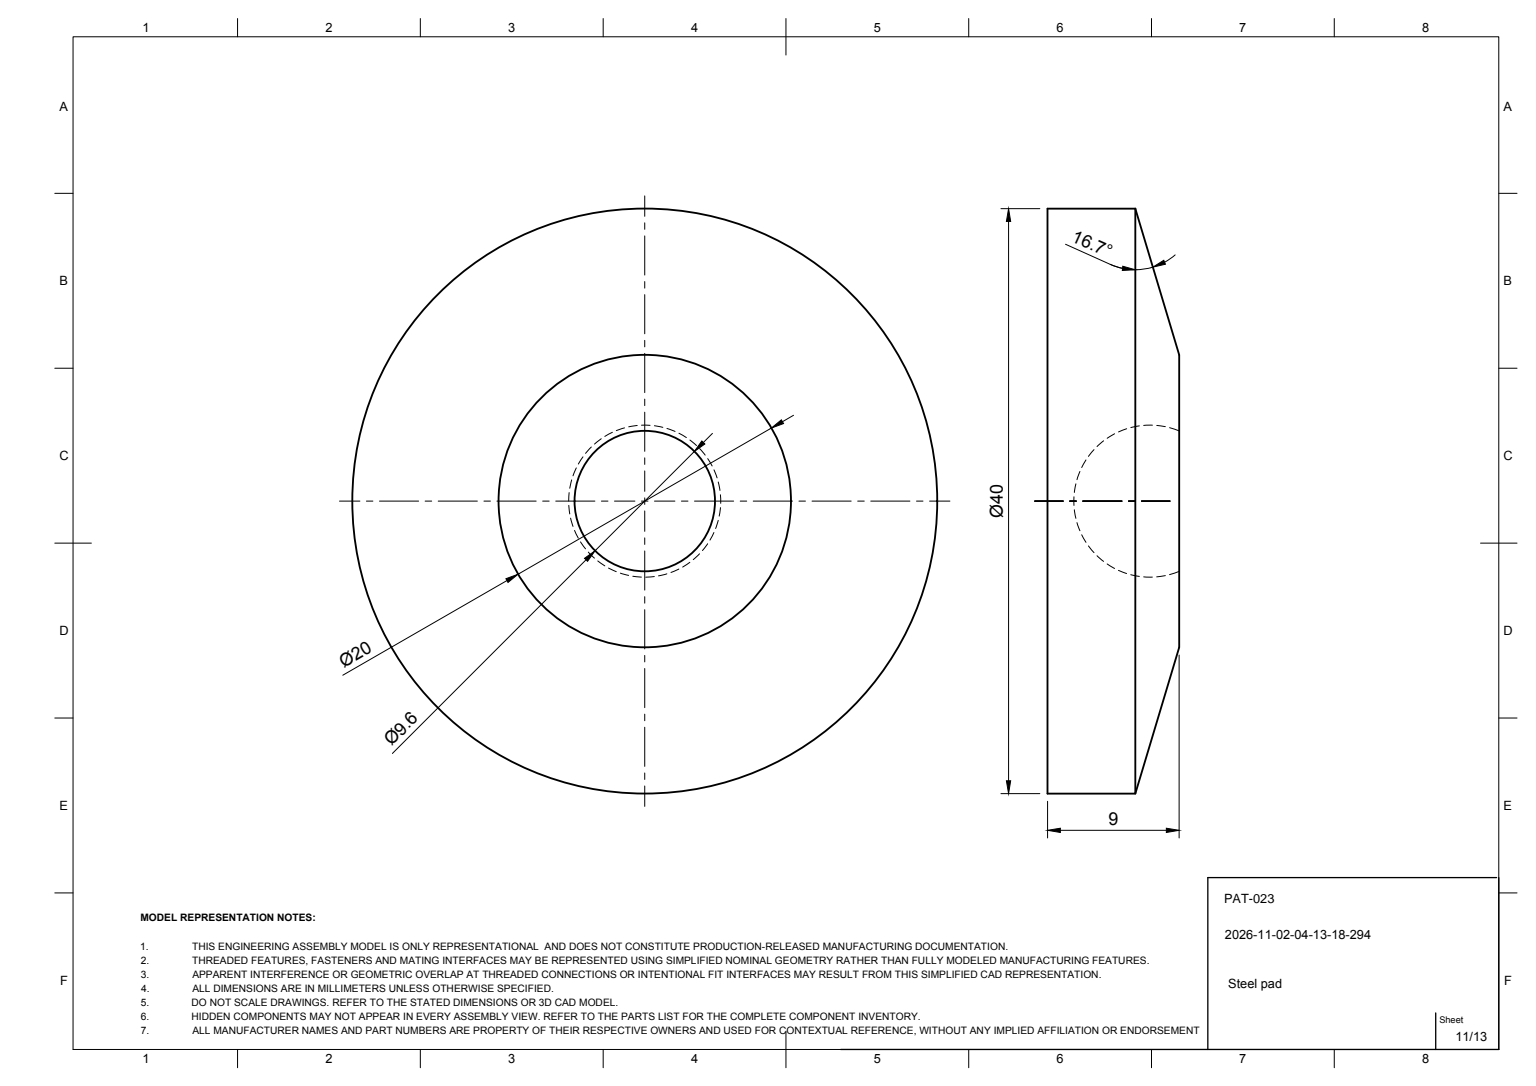
ISO-10303-21;
HEADER;
/* Generated by software containing ST-Developer
 * from STEP Tools, Inc. (www.steptools.com) 
 */

FILE_DESCRIPTION(
/* description */ ('PAT-023'),
/* implementation_level */ '2;1');

FILE_NAME(
/* name */ 'Steel pad.step',
/* time_stamp */ '2026-10-29T15:47:46-07:00',
/* author */ (''),
/* organization */ (''),
/* preprocessor_version */ 'ST-DEVELOPER v20.2',
/* originating_system */ 'Autodesk Translation Framework v15.17.0.0',
/* authorisation */ '');

FILE_SCHEMA (('AUTOMOTIVE_DESIGN { 1 0 10303 214 3 1 1 }'));
ENDSEC;

DATA;
#10=MECHANICAL_DESIGN_GEOMETRIC_PRESENTATION_REPRESENTATION('',(#88),#3773);
#61=SPHERICAL_SURFACE('',#2393,0.52);
#64=CONICAL_SURFACE('',#2400,1.5,1.27933953231703);
#72=SHAPE_REPRESENTATION_RELATIONSHIP('SRR','None',#3820,#80);
#80=ADVANCED_BREP_SHAPE_REPRESENTATION('',(#96),#3768);
#88=STYLED_ITEM('',(#3932),#96);
#96=MANIFOLD_SOLID_BREP('Body1',#2241);
#109=FACE_BOUND('',#393,.T.);
#152=PLANE('',#2396);
#153=PLANE('',#2402);
#260=FACE_OUTER_BOUND('',#388,.T.);
#261=FACE_OUTER_BOUND('',#389,.T.);
#262=FACE_OUTER_BOUND('',#390,.T.);
#263=FACE_OUTER_BOUND('',#391,.T.);
#264=FACE_OUTER_BOUND('',#392,.T.);
#388=EDGE_LOOP('',(#1721,#1722,#1723));
#389=EDGE_LOOP('',(#1724));
#390=EDGE_LOOP('',(#1725,#1726,#1727,#1728));
#391=EDGE_LOOP('',(#1729,#1730,#1731,#1732));
#392=EDGE_LOOP('',(#1733));
#393=EDGE_LOOP('',(#1734));
#564=LINE('',#3332,#828);
#565=LINE('',#3336,#829);
#828=VECTOR('',#2727,2.);
#829=VECTOR('',#2732,1.5);
#1008=CIRCLE('',#2394,0.48);
#1009=CIRCLE('',#2395,0.52);
#1010=CIRCLE('',#2397,2.);
#1011=CIRCLE('',#2399,2.);
#1012=CIRCLE('',#2401,1.);
#1092=VERTEX_POINT('',#3322);
#1093=VERTEX_POINT('',#3324);
#1094=VERTEX_POINT('',#3327);
#1095=VERTEX_POINT('',#3330);
#1096=VERTEX_POINT('',#3334);
#1323=EDGE_CURVE('',#1092,#1092,#1008,.T.);
#1324=EDGE_CURVE('',#1093,#1092,#1009,.T.);
#1325=EDGE_CURVE('',#1094,#1094,#1010,.T.);
#1326=EDGE_CURVE('',#1095,#1095,#1011,.T.);
#1327=EDGE_CURVE('',#1095,#1094,#564,.T.);
#1328=EDGE_CURVE('',#1096,#1096,#1012,.T.);
#1329=EDGE_CURVE('',#1096,#1095,#565,.T.);
#1721=ORIENTED_EDGE('',*,*,#1323,.F.);
#1722=ORIENTED_EDGE('',*,*,#1324,.F.);
#1723=ORIENTED_EDGE('',*,*,#1324,.T.);
#1724=ORIENTED_EDGE('',*,*,#1325,.F.);
#1725=ORIENTED_EDGE('',*,*,#1326,.F.);
#1726=ORIENTED_EDGE('',*,*,#1327,.T.);
#1727=ORIENTED_EDGE('',*,*,#1325,.T.);
#1728=ORIENTED_EDGE('',*,*,#1327,.F.);
#1729=ORIENTED_EDGE('',*,*,#1328,.F.);
#1730=ORIENTED_EDGE('',*,*,#1329,.T.);
#1731=ORIENTED_EDGE('',*,*,#1326,.T.);
#1732=ORIENTED_EDGE('',*,*,#1329,.F.);
#1733=ORIENTED_EDGE('',*,*,#1328,.T.);
#1734=ORIENTED_EDGE('',*,*,#1323,.T.);
#2113=CYLINDRICAL_SURFACE('',#2398,2.);
#2160=ADVANCED_FACE('',(#260),#61,.F.);
#2161=ADVANCED_FACE('',(#261),#152,.T.);
#2162=ADVANCED_FACE('',(#262),#2113,.T.);
#2163=ADVANCED_FACE('',(#263),#64,.T.);
#2164=ADVANCED_FACE('',(#264,#109),#153,.T.);
#2241=CLOSED_SHELL('',(#2160,#2161,#2162,#2163,#2164));
#2392=AXIS2_PLACEMENT_3D('',#3320,#2711,#2712);
#2393=AXIS2_PLACEMENT_3D('',#3321,#2713,#2714);
#2394=AXIS2_PLACEMENT_3D('',#3323,#2715,#2716);
#2395=AXIS2_PLACEMENT_3D('',#3325,#2717,#2718);
#2396=AXIS2_PLACEMENT_3D('',#3326,#2719,#2720);
#2397=AXIS2_PLACEMENT_3D('',#3328,#2721,#2722);
#2398=AXIS2_PLACEMENT_3D('',#3329,#2723,#2724);
#2399=AXIS2_PLACEMENT_3D('',#3331,#2725,#2726);
#2400=AXIS2_PLACEMENT_3D('',#3333,#2728,#2729);
#2401=AXIS2_PLACEMENT_3D('',#3335,#2730,#2731);
#2402=AXIS2_PLACEMENT_3D('',#3337,#2733,#2734);
#2711=DIRECTION('axis',(0.,0.,1.));
#2712=DIRECTION('refdir',(1.,0.,0.));
#2713=DIRECTION('center_axis',(6.12323399573676E-17,0.,1.));
#2714=DIRECTION('ref_axis',(1.,0.,0.));
#2715=DIRECTION('center_axis',(0.,0.,-1.));
#2716=DIRECTION('ref_axis',(0.,1.,0.));
#2717=DIRECTION('center_axis',(-1.22464679914735E-16,1.,0.));
#2718=DIRECTION('ref_axis',(-1.,-1.22464679914735E-16,0.));
#2719=DIRECTION('center_axis',(0.,0.,-1.));
#2720=DIRECTION('ref_axis',(-1.,0.,0.));
#2721=DIRECTION('center_axis',(0.,0.,1.));
#2722=DIRECTION('ref_axis',(1.,0.,0.));
#2723=DIRECTION('center_axis',(0.,0.,1.));
#2724=DIRECTION('ref_axis',(1.,0.,0.));
#2725=DIRECTION('center_axis',(0.,0.,1.));
#2726=DIRECTION('ref_axis',(1.,0.,0.));
#2727=DIRECTION('',(0.,0.,-1.));
#2728=DIRECTION('center_axis',(0.,0.,-1.));
#2729=DIRECTION('ref_axis',(1.,0.,0.));
#2730=DIRECTION('center_axis',(0.,0.,1.));
#2731=DIRECTION('ref_axis',(1.,0.,0.));
#2732=DIRECTION('',(-0.957826285221151,-1.17299889433528E-16,-0.287347885566345));
#2733=DIRECTION('center_axis',(0.,0.,1.));
#2734=DIRECTION('ref_axis',(1.,0.,0.));
#3320=CARTESIAN_POINT('',(0.,0.,0.));
#3321=CARTESIAN_POINT('Origin',(1.11022302462516E-16,0.,1.1));
#3322=CARTESIAN_POINT('',(-0.48,-5.8783046359073E-17,1.3));
#3323=CARTESIAN_POINT('Origin',(1.11022302462516E-16,0.,1.3));
#3324=CARTESIAN_POINT('',(7.91814856846845E-17,-3.89937543492083E-33,0.58));
#3325=CARTESIAN_POINT('Origin',(1.11022302462516E-16,0.,1.1));
#3326=CARTESIAN_POINT('Origin',(2.,0.,0.4));
#3327=CARTESIAN_POINT('',(-2.,-2.44929359829471E-16,0.4));
#3328=CARTESIAN_POINT('Origin',(0.,0.,0.4));
#3329=CARTESIAN_POINT('Origin',(0.,0.,0.7));
#3330=CARTESIAN_POINT('',(-2.,-2.44929359829471E-16,1.));
#3331=CARTESIAN_POINT('Origin',(0.,0.,1.));
#3332=CARTESIAN_POINT('',(-2.,-2.44929359829471E-16,0.7));
#3333=CARTESIAN_POINT('Origin',(0.,0.,1.15));
#3334=CARTESIAN_POINT('',(-1.,-1.22464679914735E-16,1.3));
#3335=CARTESIAN_POINT('Origin',(0.,0.,1.3));
#3336=CARTESIAN_POINT('',(-1.5,-1.83697019872103E-16,1.15));
#3337=CARTESIAN_POINT('Origin',(0.,0.,1.3));
#3755=UNCERTAINTY_MEASURE_WITH_UNIT(LENGTH_MEASURE(0.001),#3774,
'DISTANCE_ACCURACY_VALUE',
'Maximum model space distance between geometric entities at asserted c
onnectivities');
#3760=UNCERTAINTY_MEASURE_WITH_UNIT(LENGTH_MEASURE(0.001),#3774,
'DISTANCE_ACCURACY_VALUE',
'Maximum model space distance between geometric entities at asserted c
onnectivities');
#3768=(
GEOMETRIC_REPRESENTATION_CONTEXT(3)
GLOBAL_UNCERTAINTY_ASSIGNED_CONTEXT((#3755))
GLOBAL_UNIT_ASSIGNED_CONTEXT((#3774,#3776,#3777))
REPRESENTATION_CONTEXT('','3D')
);
#3773=(
GEOMETRIC_REPRESENTATION_CONTEXT(3)
GLOBAL_UNCERTAINTY_ASSIGNED_CONTEXT((#3760))
GLOBAL_UNIT_ASSIGNED_CONTEXT((#3774,#3776,#3777))
REPRESENTATION_CONTEXT('','3D')
);
#3774=(
LENGTH_UNIT()
NAMED_UNIT(*)
SI_UNIT(.CENTI.,.METRE.)
);
#3776=(
NAMED_UNIT(*)
PLANE_ANGLE_UNIT()
SI_UNIT($,.RADIAN.)
);
#3777=(
NAMED_UNIT(*)
SI_UNIT($,.STERADIAN.)
SOLID_ANGLE_UNIT()
);
#3785=SHAPE_DEFINITION_REPRESENTATION(#3797,#3820);
#3797=PRODUCT_DEFINITION_SHAPE('',$,#3833);
#3820=SHAPE_REPRESENTATION('',(#2392),#3768);
#3825=PRODUCT_DEFINITION_CONTEXT('part definition',#3863,'design');
#3833=PRODUCT_DEFINITION('Steel pad','Steel pad',#3845,#3825);
#3845=PRODUCT_DEFINITION_FORMATION('',$,#3872);
#3863=APPLICATION_CONTEXT(
'Core Data for Automotive Mechanical Design Process');
#3864=PRODUCT_CONTEXT('part definition',#3863,'mechanical');
#3872=PRODUCT('Steel pad','Steel pad','Steel pad',(#3864));
#3926=COLOUR_RGB('Light Blue',0.38,0.62,0.78);
#3927=FILL_AREA_STYLE_COLOUR('',#3926);
#3928=FILL_AREA_STYLE('',(#3927));
#3929=SURFACE_STYLE_FILL_AREA(#3928);
#3930=SURFACE_SIDE_STYLE('',(#3929));
#3931=SURFACE_STYLE_USAGE(.BOTH.,#3930);
#3932=PRESENTATION_STYLE_ASSIGNMENT((#3931));
ENDSEC;
END-ISO-10303-21;
